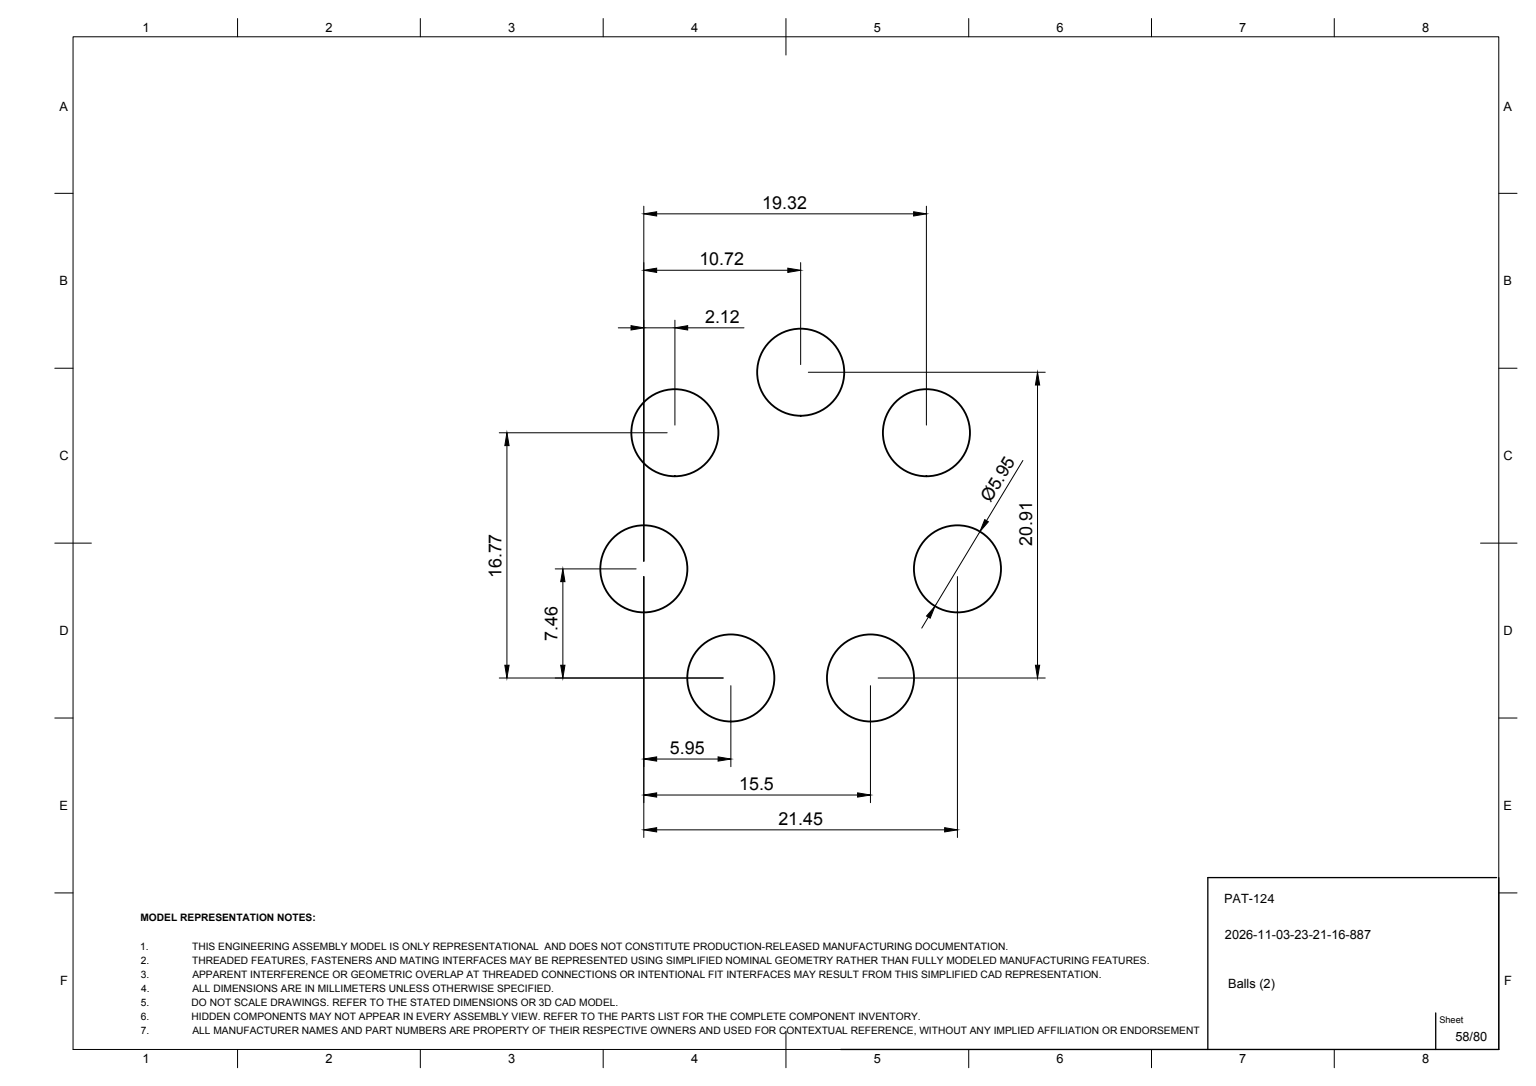
ISO-10303-21;
HEADER;
/* Generated by software containing ST-Developer
 * from STEP Tools, Inc. (www.steptools.com) 
 */

FILE_DESCRIPTION(
/* description */ ('XY cross-slide table'),
/* implementation_level */ '2;1');

FILE_NAME(
/* name */ 'Balls (2).step',
/* time_stamp */ '2026-10-28T03:22:46-07:00',
/* author */ (''),
/* organization */ (''),
/* preprocessor_version */ 'ST-DEVELOPER v20.2',
/* originating_system */ 'Autodesk Translation Framework v15.17.0.0',
/* authorisation */ '');

FILE_SCHEMA (('AUTOMOTIVE_DESIGN { 1 0 10303 214 3 1 1 }'));
ENDSEC;

DATA;
#10=MECHANICAL_DESIGN_GEOMETRIC_PRESENTATION_REPRESENTATION('',(#1738,#1739,#1740,#1741,#1742,#1743,#1744),#62984);
#1411=SPHERICAL_SURFACE('',#25572,0.29765);
#1412=SPHERICAL_SURFACE('',#25574,0.29765);
#1413=SPHERICAL_SURFACE('',#25576,0.29765);
#1414=SPHERICAL_SURFACE('',#25578,0.29765);
#1415=SPHERICAL_SURFACE('',#25580,0.29765);
#1416=SPHERICAL_SURFACE('',#25582,0.29765);
#1417=SPHERICAL_SURFACE('',#25584,0.29765);
#1557=SHAPE_REPRESENTATION_RELATIONSHIP('SRR','None',#63413,#1640);
#1640=ADVANCED_BREP_SHAPE_REPRESENTATION('',(#1847,#1848,#1849,#1850,#1851,
#1852,#1853),#62950);
#1738=STYLED_ITEM('',(#63912),#1847);
#1739=STYLED_ITEM('',(#63912),#1848);
#1740=STYLED_ITEM('',(#63912),#1849);
#1741=STYLED_ITEM('',(#63912),#1850);
#1742=STYLED_ITEM('',(#63912),#1851);
#1743=STYLED_ITEM('',(#63912),#1852);
#1744=STYLED_ITEM('',(#63912),#1853);
#1847=MANIFOLD_SOLID_BREP('Body1',#23036);
#1848=MANIFOLD_SOLID_BREP('Body2',#23037);
#1849=MANIFOLD_SOLID_BREP('Body3',#23038);
#1850=MANIFOLD_SOLID_BREP('Body4',#23039);
#1851=MANIFOLD_SOLID_BREP('Body5',#23040);
#1852=MANIFOLD_SOLID_BREP('Body6',#23041);
#1853=MANIFOLD_SOLID_BREP('Body7',#23042);
#3691=FACE_OUTER_BOUND('',#5323,.T.);
#3692=FACE_OUTER_BOUND('',#5324,.T.);
#3693=FACE_OUTER_BOUND('',#5325,.T.);
#3694=FACE_OUTER_BOUND('',#5326,.T.);
#3695=FACE_OUTER_BOUND('',#5327,.T.);
#3696=FACE_OUTER_BOUND('',#5328,.T.);
#3697=FACE_OUTER_BOUND('',#5329,.T.);
#5323=EDGE_LOOP('',(#18692,#18693));
#5324=EDGE_LOOP('',(#18694,#18695));
#5325=EDGE_LOOP('',(#18696,#18697));
#5326=EDGE_LOOP('',(#18698,#18699));
#5327=EDGE_LOOP('',(#18700,#18701));
#5328=EDGE_LOOP('',(#18702,#18703));
#5329=EDGE_LOOP('',(#18704,#18705));
#9489=CIRCLE('',#25573,0.29765);
#9490=CIRCLE('',#25575,0.29765);
#9491=CIRCLE('',#25577,0.29765);
#9492=CIRCLE('',#25579,0.29765);
#9493=CIRCLE('',#25581,0.29765);
#9494=CIRCLE('',#25583,0.29765);
#9495=CIRCLE('',#25585,0.29765);
#11041=VERTEX_POINT('',#48605);
#11042=VERTEX_POINT('',#48606);
#11043=VERTEX_POINT('',#48609);
#11044=VERTEX_POINT('',#48610);
#11045=VERTEX_POINT('',#48613);
#11046=VERTEX_POINT('',#48614);
#11047=VERTEX_POINT('',#48617);
#11048=VERTEX_POINT('',#48618);
#11049=VERTEX_POINT('',#48621);
#11050=VERTEX_POINT('',#48622);
#11051=VERTEX_POINT('',#48625);
#11052=VERTEX_POINT('',#48626);
#11053=VERTEX_POINT('',#48629);
#11054=VERTEX_POINT('',#48630);
#13730=EDGE_CURVE('',#11041,#11042,#9489,.T.);
#13731=EDGE_CURVE('',#11043,#11044,#9490,.T.);
#13732=EDGE_CURVE('',#11045,#11046,#9491,.T.);
#13733=EDGE_CURVE('',#11047,#11048,#9492,.T.);
#13734=EDGE_CURVE('',#11049,#11050,#9493,.T.);
#13735=EDGE_CURVE('',#11051,#11052,#9494,.T.);
#13736=EDGE_CURVE('',#11053,#11054,#9495,.T.);
#18692=ORIENTED_EDGE('',*,*,#13730,.T.);
#18693=ORIENTED_EDGE('',*,*,#13730,.F.);
#18694=ORIENTED_EDGE('',*,*,#13731,.T.);
#18695=ORIENTED_EDGE('',*,*,#13731,.F.);
#18696=ORIENTED_EDGE('',*,*,#13732,.T.);
#18697=ORIENTED_EDGE('',*,*,#13732,.F.);
#18698=ORIENTED_EDGE('',*,*,#13733,.T.);
#18699=ORIENTED_EDGE('',*,*,#13733,.F.);
#18700=ORIENTED_EDGE('',*,*,#13734,.T.);
#18701=ORIENTED_EDGE('',*,*,#13734,.F.);
#18702=ORIENTED_EDGE('',*,*,#13735,.T.);
#18703=ORIENTED_EDGE('',*,*,#13735,.F.);
#18704=ORIENTED_EDGE('',*,*,#13736,.T.);
#18705=ORIENTED_EDGE('',*,*,#13736,.F.);
#22472=ADVANCED_FACE('',(#3691),#1411,.T.);
#22473=ADVANCED_FACE('',(#3692),#1412,.T.);
#22474=ADVANCED_FACE('',(#3693),#1413,.T.);
#22475=ADVANCED_FACE('',(#3694),#1414,.T.);
#22476=ADVANCED_FACE('',(#3695),#1415,.T.);
#22477=ADVANCED_FACE('',(#3696),#1416,.T.);
#22478=ADVANCED_FACE('',(#3697),#1417,.T.);
#23036=CLOSED_SHELL('',(#22472));
#23037=CLOSED_SHELL('',(#22473));
#23038=CLOSED_SHELL('',(#22474));
#23039=CLOSED_SHELL('',(#22475));
#23040=CLOSED_SHELL('',(#22476));
#23041=CLOSED_SHELL('',(#22477));
#23042=CLOSED_SHELL('',(#22478));
#25571=AXIS2_PLACEMENT_3D('',#48603,#30544,#30545);
#25572=AXIS2_PLACEMENT_3D('',#48604,#30546,#30547);
#25573=AXIS2_PLACEMENT_3D('',#48607,#30548,#30549);
#25574=AXIS2_PLACEMENT_3D('',#48608,#30550,#30551);
#25575=AXIS2_PLACEMENT_3D('',#48611,#30552,#30553);
#25576=AXIS2_PLACEMENT_3D('',#48612,#30554,#30555);
#25577=AXIS2_PLACEMENT_3D('',#48615,#30556,#30557);
#25578=AXIS2_PLACEMENT_3D('',#48616,#30558,#30559);
#25579=AXIS2_PLACEMENT_3D('',#48619,#30560,#30561);
#25580=AXIS2_PLACEMENT_3D('',#48620,#30562,#30563);
#25581=AXIS2_PLACEMENT_3D('',#48623,#30564,#30565);
#25582=AXIS2_PLACEMENT_3D('',#48624,#30566,#30567);
#25583=AXIS2_PLACEMENT_3D('',#48627,#30568,#30569);
#25584=AXIS2_PLACEMENT_3D('',#48628,#30570,#30571);
#25585=AXIS2_PLACEMENT_3D('',#48631,#30572,#30573);
#30544=DIRECTION('axis',(0.,0.,1.));
#30545=DIRECTION('refdir',(1.,0.,0.));
#30546=DIRECTION('center_axis',(0.,0.,1.));
#30547=DIRECTION('ref_axis',(1.,0.,0.));
#30548=DIRECTION('center_axis',(1.22464679914735E-16,-1.,0.));
#30549=DIRECTION('ref_axis',(-1.,-1.22464679914735E-16,0.));
#30550=DIRECTION('center_axis',(0.78183148246803,0.,0.623489801858733));
#30551=DIRECTION('ref_axis',(0.623489801858734,0.,-0.78183148246803));
#30552=DIRECTION('center_axis',(7.63554790147315E-17,-1.,-9.57467422477103E-17));
#30553=DIRECTION('ref_axis',(-0.623489801858734,-1.22464679914735E-16,0.78183148246803));
#30554=DIRECTION('center_axis',(0.974927912181824,0.,-0.222520933956314));
#30555=DIRECTION('ref_axis',(-0.222520933956314,0.,-0.974927912181824));
#30556=DIRECTION('center_axis',(-2.7250954951288E-17,-1.,-1.19394234705288E-16));
#30557=DIRECTION('ref_axis',(0.222520933956314,-1.22464679914735E-16,0.974927912181824));
#30558=DIRECTION('center_axis',(0.433883739117558,0.,-0.900968867902419));
#30559=DIRECTION('ref_axis',(-0.900968867902419,0.,-0.433883739117558));
#30560=DIRECTION('center_axis',(-1.10336864020811E-16,-1.,-5.31354332312403E-17));
#30561=DIRECTION('ref_axis',(0.900968867902419,-1.22464679914735E-16,0.433883739117558));
#30562=DIRECTION('center_axis',(-0.433883739117558,0.,-0.900968867902419));
#30563=DIRECTION('ref_axis',(-0.900968867902419,0.,0.433883739117558));
#30564=DIRECTION('center_axis',(-1.10336864020811E-16,-1.,5.31354332312403E-17));
#30565=DIRECTION('ref_axis',(0.900968867902419,-1.22464679914735E-16,-0.433883739117558));
#30566=DIRECTION('center_axis',(-0.974927912181824,0.,-0.222520933956314));
#30567=DIRECTION('ref_axis',(-0.222520933956315,0.,0.974927912181824));
#30568=DIRECTION('center_axis',(-2.7250954951288E-17,-1.,1.19394234705288E-16));
#30569=DIRECTION('ref_axis',(0.222520933956315,-1.22464679914735E-16,-0.974927912181824));
#30570=DIRECTION('center_axis',(-0.78183148246803,0.,0.623489801858734));
#30571=DIRECTION('ref_axis',(0.623489801858733,0.,0.78183148246803));
#30572=DIRECTION('center_axis',(7.63554790147315E-17,-1.,9.57467422477103E-17));
#30573=DIRECTION('ref_axis',(-0.623489801858733,-1.22464679914735E-16,-0.78183148246803));
#48603=CARTESIAN_POINT('',(0.,0.,0.));
#48604=CARTESIAN_POINT('Origin',(1.1,0.,0.));
#48605=CARTESIAN_POINT('',(1.1,-2.23201749654651E-33,0.29765));
#48606=CARTESIAN_POINT('',(1.1,-2.23201749654651E-33,-0.29765));
#48607=CARTESIAN_POINT('Origin',(1.1,0.,0.));
#48608=CARTESIAN_POINT('Origin',(0.685838782044607,0.,-0.860014630714833));
#48609=CARTESIAN_POINT('',(0.918550922801216,-5.31350540756609E-33,-0.674432891191581));
#48610=CARTESIAN_POINT('',(0.453126641287998,8.49470414473068E-34,-1.04559637023808));
#48611=CARTESIAN_POINT('Origin',(0.685838782044607,0.,-0.860014630714833));
#48612=CARTESIAN_POINT('Origin',(-0.244773027351946,0.,-1.07242070340001));
#48613=CARTESIAN_POINT('',(0.0454142657089739,-2.23201749654651E-33,-1.1386540593921));
#48614=CARTESIAN_POINT('',(-0.534960320412865,-2.23201749654651E-33,-1.00618734740791));
#48615=CARTESIAN_POINT('Origin',(-0.244773027351946,0.,-1.07242070340001));
#48616=CARTESIAN_POINT('Origin',(-0.991065754692661,0.,-0.477272113029314));
#48617=CARTESIAN_POINT('',(-0.86192025974432,8.49470414473067E-34,-0.745445496560469));
#48618=CARTESIAN_POINT('',(-1.120211249641,-5.31350540756609E-33,-0.209098729498159));
#48619=CARTESIAN_POINT('Origin',(-0.991065754692661,0.,-0.477272113029314));
#48620=CARTESIAN_POINT('Origin',(-0.991065754692661,0.,0.477272113029314));
#48621=CARTESIAN_POINT('',(-1.120211249641,-2.23201749654651E-33,0.209098729498159));
#48622=CARTESIAN_POINT('',(-0.86192025974432,-2.23201749654651E-33,0.745445496560469));
#48623=CARTESIAN_POINT('Origin',(-0.991065754692661,0.,0.477272113029314));
#48624=CARTESIAN_POINT('Origin',(-0.244773027351946,0.,1.07242070340001));
#48625=CARTESIAN_POINT('',(-0.534960320412866,-2.23201749654651E-33,1.00618734740791));
#48626=CARTESIAN_POINT('',(0.0454142657089737,-2.23201749654651E-33,1.1386540593921));
#48627=CARTESIAN_POINT('Origin',(-0.244773027351946,0.,1.07242070340001));
#48628=CARTESIAN_POINT('Origin',(0.685838782044607,0.,0.860014630714833));
#48629=CARTESIAN_POINT('',(0.453126641287998,-2.23201749654651E-33,1.04559637023808));
#48630=CARTESIAN_POINT('',(0.918550922801216,-2.23201749654651E-33,0.674432891191581));
#48631=CARTESIAN_POINT('Origin',(0.685838782044607,0.,0.860014630714833));
#62851=UNCERTAINTY_MEASURE_WITH_UNIT(LENGTH_MEASURE(0.001),#62985,
'DISTANCE_ACCURACY_VALUE',
'Maximum model space distance between geometric entities at asserted c
onnectivities');
#62885=UNCERTAINTY_MEASURE_WITH_UNIT(LENGTH_MEASURE(0.001),#62985,
'DISTANCE_ACCURACY_VALUE',
'Maximum model space distance between geometric entities at asserted c
onnectivities');
#62950=(
GEOMETRIC_REPRESENTATION_CONTEXT(3)
GLOBAL_UNCERTAINTY_ASSIGNED_CONTEXT((#62851))
GLOBAL_UNIT_ASSIGNED_CONTEXT((#62985,#62987,#62988))
REPRESENTATION_CONTEXT('','3D')
);
#62984=(
GEOMETRIC_REPRESENTATION_CONTEXT(3)
GLOBAL_UNCERTAINTY_ASSIGNED_CONTEXT((#62885))
GLOBAL_UNIT_ASSIGNED_CONTEXT((#62985,#62987,#62988))
REPRESENTATION_CONTEXT('','3D')
);
#62985=(
LENGTH_UNIT()
NAMED_UNIT(*)
SI_UNIT(.CENTI.,.METRE.)
);
#62987=(
NAMED_UNIT(*)
PLANE_ANGLE_UNIT()
SI_UNIT($,.RADIAN.)
);
#62988=(
NAMED_UNIT(*)
SI_UNIT($,.STERADIAN.)
SOLID_ANGLE_UNIT()
);
#63053=SHAPE_DEFINITION_REPRESENTATION(#63231,#63413);
#63231=PRODUCT_DEFINITION_SHAPE('',$,#63512);
#63413=SHAPE_REPRESENTATION('',(#25571),#62950);
#63447=PRODUCT_DEFINITION_CONTEXT('part definition',#63743,'design');
#63512=PRODUCT_DEFINITION('Balls (2)','Balls (2)',#63610,#63447);
#63610=PRODUCT_DEFINITION_FORMATION('',$,#63809);
#63743=APPLICATION_CONTEXT(
'Core Data for Automotive Mechanical Design Process');
#63744=PRODUCT_CONTEXT('part definition',#63743,'mechanical');
#63809=PRODUCT('Balls (2)','Balls (2)','Balls (2)',(#63744));
#63906=COLOUR_RGB('Grey',0.48,0.52,0.57);
#63907=FILL_AREA_STYLE_COLOUR('',#63906);
#63908=FILL_AREA_STYLE('',(#63907));
#63909=SURFACE_STYLE_FILL_AREA(#63908);
#63910=SURFACE_SIDE_STYLE('',(#63909));
#63911=SURFACE_STYLE_USAGE(.BOTH.,#63910);
#63912=PRESENTATION_STYLE_ASSIGNMENT((#63911));
ENDSEC;
END-ISO-10303-21;
